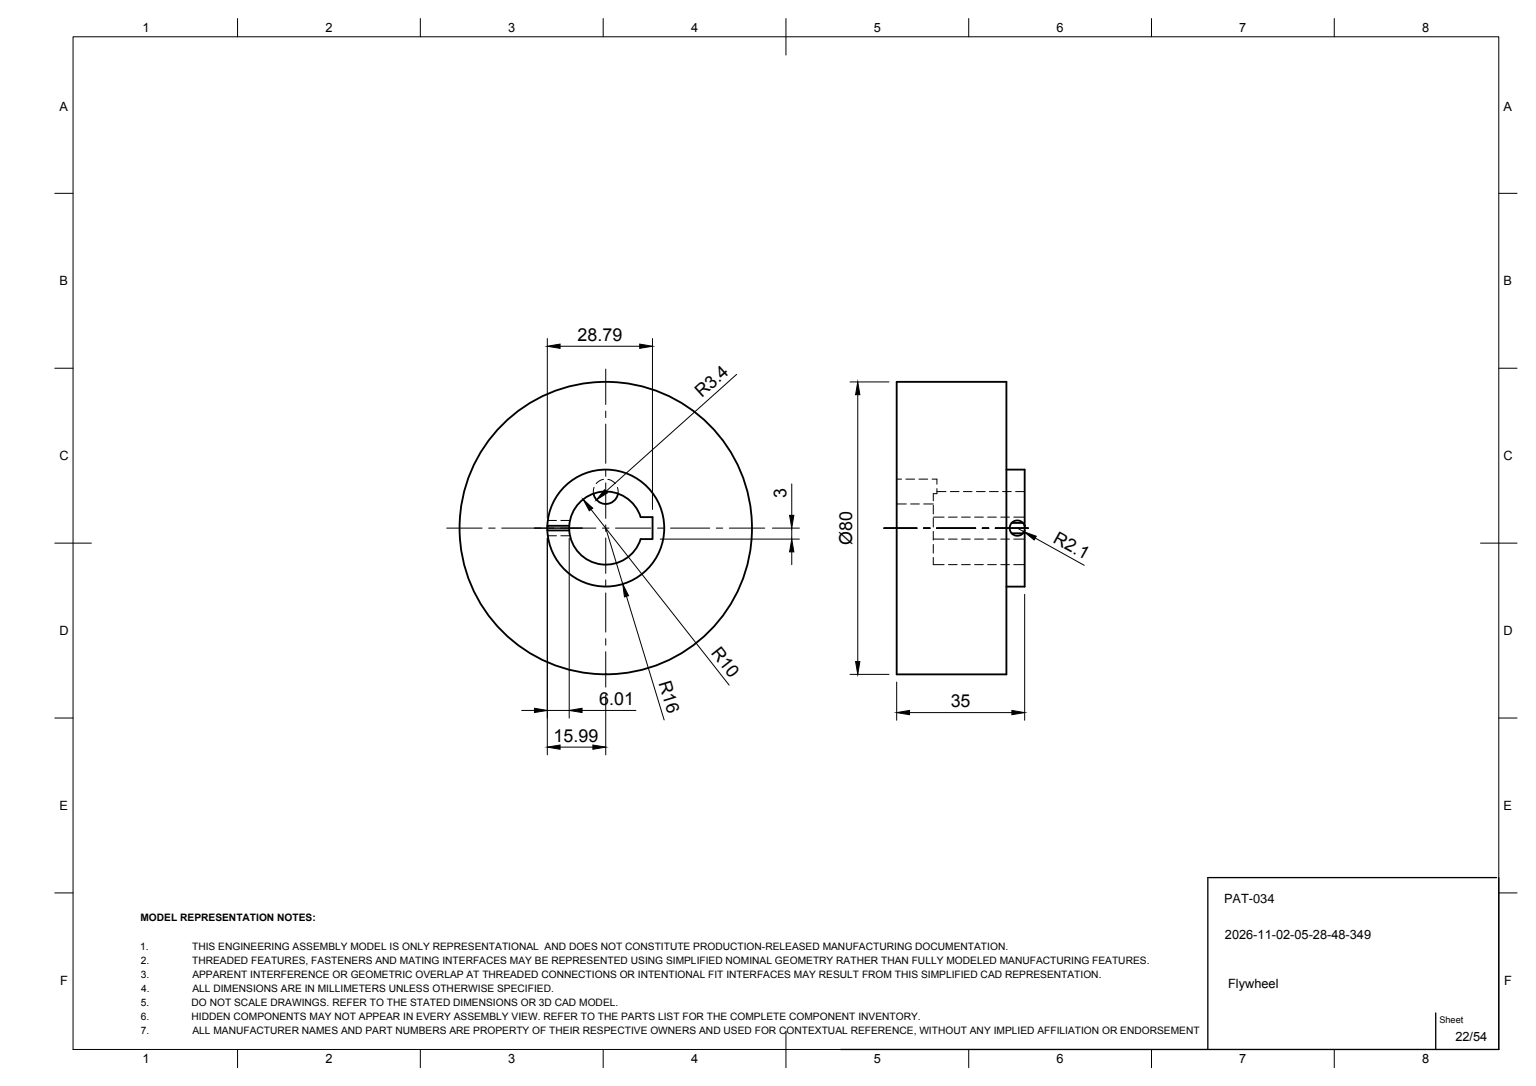
ISO-10303-21;
HEADER;
/* Generated by software containing ST-Developer
 * from STEP Tools, Inc. (www.steptools.com) 
 */

FILE_DESCRIPTION(
/* description */ ('Fatigue rig crank-slider'),
/* implementation_level */ '2;1');

FILE_NAME(
/* name */ 'Flywheel.step',
/* time_stamp */ '2026-10-28T03:24:50-07:00',
/* author */ (''),
/* organization */ (''),
/* preprocessor_version */ 'ST-DEVELOPER v20.2',
/* originating_system */ 'Autodesk Translation Framework v15.17.0.0',
/* authorisation */ '');

FILE_SCHEMA (('AUTOMOTIVE_DESIGN { 1 0 10303 214 3 1 1 }'));
ENDSEC;

DATA;
#10=MECHANICAL_DESIGN_GEOMETRIC_PRESENTATION_REPRESENTATION('',(#608),#16911);
#447=B_SPLINE_CURVE_WITH_KNOTS('',3,(#15046,#15047,#15048,#15049,#15050,
#15051),.UNSPECIFIED.,.F.,.F.,(4,2,4),(1.01510699658258,1.03166343394832,
1.10079263710785),.UNSPECIFIED.);
#448=B_SPLINE_CURVE_WITH_KNOTS('',3,(#15055,#15056,#15057,#15058,#15059,
#15060,#15061,#15062,#15063,#15064),.UNSPECIFIED.,.F.,.F.,(4,2,2,2,4),(0.168950313426779,
0.238079516586307,0.317435737633656,0.396791958681006,0.465921161840534),
 .UNSPECIFIED.);
#449=B_SPLINE_CURVE_WITH_KNOTS('',3,(#15068,#15069,#15070,#15071,#15072,
#15073),.UNSPECIFIED.,.F.,.F.,(4,2,4),(0.803821788694091,0.872950991853619,
0.88950742921936),.UNSPECIFIED.);
#450=B_SPLINE_CURVE_WITH_KNOTS('',3,(#15103,#15104,#15105,#15106,#15107,
#15108,#15109,#15110,#15111,#15112,#15113,#15114,#15115,#15116,#15117,#15118,
#15119,#15120,#15121,#15122,#15123,#15124,#15125,#15126,#15127,#15128,#15129,
#15130,#15131,#15132,#15133,#15134,#15135,#15136,#15137),.UNSPECIFIED.,
 .F.,.F.,(4,2,2,2,2,2,2,2,2,2,2,2,3,2,2,2,4),(0.379554434981269,0.396011596624156,
0.475213593758045,0.554416396369289,0.633619198980533,0.712822001591777,
0.792024804203021,0.87122680133691,0.950428798470799,1.02963079560469,1.10883279273858,
1.18803559534982,1.26723839796107,1.34644120057231,1.42564400318355,1.50484600031744,
1.52130316196033),.UNSPECIFIED.);
#507=SHAPE_REPRESENTATION_RELATIONSHIP('SRR','None',#17148,#557);
#557=ADVANCED_BREP_SHAPE_REPRESENTATION('',(#665),#16877);
#608=STYLED_ITEM('',(#17501),#665);
#665=MANIFOLD_SOLID_BREP('Body1',#8901);
#831=FACE_BOUND('',#2121,.T.);
#832=FACE_BOUND('',#2129,.T.);
#1043=PLANE('',#9952);
#1044=PLANE('',#9964);
#1045=PLANE('',#9965);
#1046=PLANE('',#9967);
#1047=PLANE('',#9968);
#1048=PLANE('',#9969);
#1049=PLANE('',#9973);
#1050=PLANE('',#9974);
#1051=PLANE('',#9975);
#1052=PLANE('',#9982);
#1462=FACE_OUTER_BOUND('',#2116,.T.);
#1463=FACE_OUTER_BOUND('',#2117,.T.);
#1464=FACE_OUTER_BOUND('',#2118,.T.);
#1465=FACE_OUTER_BOUND('',#2119,.T.);
#1466=FACE_OUTER_BOUND('',#2120,.T.);
#1467=FACE_OUTER_BOUND('',#2122,.T.);
#1468=FACE_OUTER_BOUND('',#2123,.T.);
#1469=FACE_OUTER_BOUND('',#2124,.T.);
#1470=FACE_OUTER_BOUND('',#2125,.T.);
#1471=FACE_OUTER_BOUND('',#2126,.T.);
#1472=FACE_OUTER_BOUND('',#2127,.T.);
#1473=FACE_OUTER_BOUND('',#2128,.T.);
#1474=FACE_OUTER_BOUND('',#2130,.T.);
#1475=FACE_OUTER_BOUND('',#2131,.T.);
#1476=FACE_OUTER_BOUND('',#2132,.T.);
#2116=EDGE_LOOP('',(#7026,#7027));
#2117=EDGE_LOOP('',(#7028,#7029,#7030,#7031,#7032,#7033,#7034,#7035));
#2118=EDGE_LOOP('',(#7036,#7037,#7038,#7039,#7040,#7041,#7042,#7043,#7044,
#7045,#7046,#7047,#7048,#7049));
#2119=EDGE_LOOP('',(#7050,#7051,#7052,#7053,#7054,#7055,#7056));
#2120=EDGE_LOOP('',(#7057));
#2121=EDGE_LOOP('',(#7058));
#2122=EDGE_LOOP('',(#7059,#7060,#7061,#7062));
#2123=EDGE_LOOP('',(#7063,#7064,#7065,#7066));
#2124=EDGE_LOOP('',(#7067,#7068));
#2125=EDGE_LOOP('',(#7069,#7070,#7071,#7072,#7073,#7074,#7075,#7076));
#2126=EDGE_LOOP('',(#7077,#7078));
#2127=EDGE_LOOP('',(#7079,#7080,#7081,#7082));
#2128=EDGE_LOOP('',(#7083));
#2129=EDGE_LOOP('',(#7084));
#2130=EDGE_LOOP('',(#7085,#7086,#7087,#7088));
#2131=EDGE_LOOP('',(#7089,#7090,#7091,#7092,#7093,#7094));
#2132=EDGE_LOOP('',(#7095,#7096,#7097,#7098,#7099,#7100,#7101,#7102,#7103));
#2756=LINE('',#15029,#3402);
#2757=LINE('',#15033,#3403);
#2758=LINE('',#15037,#3404);
#2759=LINE('',#15042,#3405);
#2760=LINE('',#15053,#3406);
#2761=LINE('',#15066,#3407);
#2762=LINE('',#15077,#3408);
#2763=LINE('',#15081,#3409);
#2764=LINE('',#15083,#3410);
#2765=LINE('',#15084,#3411);
#2766=LINE('',#15090,#3412);
#2767=LINE('',#15092,#3413);
#2768=LINE('',#15093,#3414);
#2769=LINE('',#15095,#3415);
#2770=LINE('',#15101,#3416);
#2771=LINE('',#15138,#3417);
#2772=LINE('',#15141,#3418);
#2773=LINE('',#15148,#3419);
#2774=LINE('',#15151,#3420);
#3402=VECTOR('',#11788,1.);
#3403=VECTOR('',#11791,0.34);
#3404=VECTOR('',#11796,1.);
#3405=VECTOR('',#11801,1.);
#3406=VECTOR('',#11804,1.);
#3407=VECTOR('',#11805,1.);
#3408=VECTOR('',#11808,1.);
#3409=VECTOR('',#11813,1.);
#3410=VECTOR('',#11814,1.);
#3411=VECTOR('',#11815,1.);
#3412=VECTOR('',#11822,1.);
#3413=VECTOR('',#11823,1.);
#3414=VECTOR('',#11824,1.);
#3415=VECTOR('',#11827,1.);
#3416=VECTOR('',#11836,1.);
#3417=VECTOR('',#11837,1.);
#3418=VECTOR('',#11842,1.);
#3419=VECTOR('',#11851,4.);
#3420=VECTOR('',#11854,1.6);
#3939=CIRCLE('',#9953,1.);
#3940=CIRCLE('',#9954,0.34);
#3941=CIRCLE('',#9956,0.34);
#3942=CIRCLE('',#9957,0.34);
#3943=CIRCLE('',#9958,0.34);
#3944=CIRCLE('',#9960,1.);
#3945=CIRCLE('',#9961,1.);
#3946=CIRCLE('',#9962,1.);
#3947=CIRCLE('',#9963,1.);
#3948=CIRCLE('',#9966,4.);
#3949=CIRCLE('',#9970,0.21);
#3950=CIRCLE('',#9972,0.21);
#3951=CIRCLE('',#9976,4.);
#3952=CIRCLE('',#9977,1.6);
#3953=CIRCLE('',#9980,1.6);
#3954=CIRCLE('',#9981,1.6);
#4501=VERTEX_POINT('',#15023);
#4502=VERTEX_POINT('',#15024);
#4503=VERTEX_POINT('',#15028);
#4504=VERTEX_POINT('',#15030);
#4505=VERTEX_POINT('',#15032);
#4506=VERTEX_POINT('',#15035);
#4507=VERTEX_POINT('',#15039);
#4508=VERTEX_POINT('',#15041);
#4509=VERTEX_POINT('',#15043);
#4510=VERTEX_POINT('',#15045);
#4511=VERTEX_POINT('',#15052);
#4512=VERTEX_POINT('',#15054);
#4513=VERTEX_POINT('',#15065);
#4514=VERTEX_POINT('',#15067);
#4515=VERTEX_POINT('',#15074);
#4516=VERTEX_POINT('',#15076);
#4517=VERTEX_POINT('',#15080);
#4518=VERTEX_POINT('',#15082);
#4519=VERTEX_POINT('',#15086);
#4520=VERTEX_POINT('',#15089);
#4521=VERTEX_POINT('',#15091);
#4522=VERTEX_POINT('',#15100);
#4523=VERTEX_POINT('',#15102);
#4524=VERTEX_POINT('',#15143);
#4525=VERTEX_POINT('',#15145);
#4526=VERTEX_POINT('',#15150);
#5411=EDGE_CURVE('',#4501,#4502,#3939,.T.);
#5412=EDGE_CURVE('',#4501,#4502,#3940,.T.);
#5413=EDGE_CURVE('',#4503,#4501,#2756,.T.);
#5414=EDGE_CURVE('',#4504,#4503,#3941,.T.);
#5415=EDGE_CURVE('',#4504,#4505,#2757,.T.);
#5416=EDGE_CURVE('',#4505,#4505,#3942,.T.);
#5417=EDGE_CURVE('',#4506,#4504,#3943,.T.);
#5418=EDGE_CURVE('',#4502,#4506,#2758,.T.);
#5419=EDGE_CURVE('',#4506,#4507,#3944,.T.);
#5420=EDGE_CURVE('',#4507,#4508,#2759,.T.);
#5421=EDGE_CURVE('',#4508,#4509,#3945,.T.);
#5422=EDGE_CURVE('',#4509,#4510,#447,.T.);
#5423=EDGE_CURVE('',#4510,#4511,#2760,.T.);
#5424=EDGE_CURVE('',#4511,#4512,#448,.T.);
#5425=EDGE_CURVE('',#4512,#4513,#2761,.T.);
#5426=EDGE_CURVE('',#4513,#4514,#449,.T.);
#5427=EDGE_CURVE('',#4514,#4515,#3946,.T.);
#5428=EDGE_CURVE('',#4515,#4516,#2762,.T.);
#5429=EDGE_CURVE('',#4516,#4503,#3947,.T.);
#5430=EDGE_CURVE('',#4517,#4516,#2763,.T.);
#5431=EDGE_CURVE('',#4518,#4517,#2764,.T.);
#5432=EDGE_CURVE('',#4507,#4518,#2765,.T.);
#5433=EDGE_CURVE('',#4519,#4519,#3948,.T.);
#5434=EDGE_CURVE('',#4520,#4517,#2766,.T.);
#5435=EDGE_CURVE('',#4521,#4520,#2767,.T.);
#5436=EDGE_CURVE('',#4521,#4518,#2768,.T.);
#5437=EDGE_CURVE('',#4520,#4515,#2769,.T.);
#5438=EDGE_CURVE('',#4512,#4513,#3949,.T.);
#5439=EDGE_CURVE('',#4510,#4511,#3950,.T.);
#5440=EDGE_CURVE('',#4522,#4509,#2770,.T.);
#5441=EDGE_CURVE('',#4523,#4522,#450,.T.);
#5442=EDGE_CURVE('',#4514,#4523,#2771,.T.);
#5443=EDGE_CURVE('',#4508,#4521,#2772,.T.);
#5444=EDGE_CURVE('',#4524,#4524,#3951,.T.);
#5445=EDGE_CURVE('',#4525,#4525,#3952,.T.);
#5446=EDGE_CURVE('',#4519,#4524,#2773,.T.);
#5447=EDGE_CURVE('',#4525,#4526,#2774,.T.);
#5448=EDGE_CURVE('',#4526,#4523,#3953,.T.);
#5449=EDGE_CURVE('',#4522,#4526,#3954,.T.);
#7026=ORIENTED_EDGE('',*,*,#5411,.F.);
#7027=ORIENTED_EDGE('',*,*,#5412,.T.);
#7028=ORIENTED_EDGE('',*,*,#5413,.F.);
#7029=ORIENTED_EDGE('',*,*,#5414,.F.);
#7030=ORIENTED_EDGE('',*,*,#5415,.T.);
#7031=ORIENTED_EDGE('',*,*,#5416,.F.);
#7032=ORIENTED_EDGE('',*,*,#5415,.F.);
#7033=ORIENTED_EDGE('',*,*,#5417,.F.);
#7034=ORIENTED_EDGE('',*,*,#5418,.F.);
#7035=ORIENTED_EDGE('',*,*,#5412,.F.);
#7036=ORIENTED_EDGE('',*,*,#5413,.T.);
#7037=ORIENTED_EDGE('',*,*,#5411,.T.);
#7038=ORIENTED_EDGE('',*,*,#5418,.T.);
#7039=ORIENTED_EDGE('',*,*,#5419,.T.);
#7040=ORIENTED_EDGE('',*,*,#5420,.T.);
#7041=ORIENTED_EDGE('',*,*,#5421,.T.);
#7042=ORIENTED_EDGE('',*,*,#5422,.T.);
#7043=ORIENTED_EDGE('',*,*,#5423,.T.);
#7044=ORIENTED_EDGE('',*,*,#5424,.T.);
#7045=ORIENTED_EDGE('',*,*,#5425,.T.);
#7046=ORIENTED_EDGE('',*,*,#5426,.T.);
#7047=ORIENTED_EDGE('',*,*,#5427,.T.);
#7048=ORIENTED_EDGE('',*,*,#5428,.T.);
#7049=ORIENTED_EDGE('',*,*,#5429,.T.);
#7050=ORIENTED_EDGE('',*,*,#5417,.T.);
#7051=ORIENTED_EDGE('',*,*,#5414,.T.);
#7052=ORIENTED_EDGE('',*,*,#5429,.F.);
#7053=ORIENTED_EDGE('',*,*,#5430,.F.);
#7054=ORIENTED_EDGE('',*,*,#5431,.F.);
#7055=ORIENTED_EDGE('',*,*,#5432,.F.);
#7056=ORIENTED_EDGE('',*,*,#5419,.F.);
#7057=ORIENTED_EDGE('',*,*,#5433,.T.);
#7058=ORIENTED_EDGE('',*,*,#5416,.T.);
#7059=ORIENTED_EDGE('',*,*,#5431,.T.);
#7060=ORIENTED_EDGE('',*,*,#5434,.F.);
#7061=ORIENTED_EDGE('',*,*,#5435,.F.);
#7062=ORIENTED_EDGE('',*,*,#5436,.T.);
#7063=ORIENTED_EDGE('',*,*,#5430,.T.);
#7064=ORIENTED_EDGE('',*,*,#5428,.F.);
#7065=ORIENTED_EDGE('',*,*,#5437,.F.);
#7066=ORIENTED_EDGE('',*,*,#5434,.T.);
#7067=ORIENTED_EDGE('',*,*,#5425,.F.);
#7068=ORIENTED_EDGE('',*,*,#5438,.T.);
#7069=ORIENTED_EDGE('',*,*,#5424,.F.);
#7070=ORIENTED_EDGE('',*,*,#5439,.F.);
#7071=ORIENTED_EDGE('',*,*,#5422,.F.);
#7072=ORIENTED_EDGE('',*,*,#5440,.F.);
#7073=ORIENTED_EDGE('',*,*,#5441,.F.);
#7074=ORIENTED_EDGE('',*,*,#5442,.F.);
#7075=ORIENTED_EDGE('',*,*,#5426,.F.);
#7076=ORIENTED_EDGE('',*,*,#5438,.F.);
#7077=ORIENTED_EDGE('',*,*,#5423,.F.);
#7078=ORIENTED_EDGE('',*,*,#5439,.T.);
#7079=ORIENTED_EDGE('',*,*,#5432,.T.);
#7080=ORIENTED_EDGE('',*,*,#5436,.F.);
#7081=ORIENTED_EDGE('',*,*,#5443,.F.);
#7082=ORIENTED_EDGE('',*,*,#5420,.F.);
#7083=ORIENTED_EDGE('',*,*,#5444,.F.);
#7084=ORIENTED_EDGE('',*,*,#5445,.F.);
#7085=ORIENTED_EDGE('',*,*,#5433,.F.);
#7086=ORIENTED_EDGE('',*,*,#5446,.T.);
#7087=ORIENTED_EDGE('',*,*,#5444,.T.);
#7088=ORIENTED_EDGE('',*,*,#5446,.F.);
#7089=ORIENTED_EDGE('',*,*,#5445,.T.);
#7090=ORIENTED_EDGE('',*,*,#5447,.T.);
#7091=ORIENTED_EDGE('',*,*,#5448,.T.);
#7092=ORIENTED_EDGE('',*,*,#5441,.T.);
#7093=ORIENTED_EDGE('',*,*,#5449,.T.);
#7094=ORIENTED_EDGE('',*,*,#5447,.F.);
#7095=ORIENTED_EDGE('',*,*,#5440,.T.);
#7096=ORIENTED_EDGE('',*,*,#5421,.F.);
#7097=ORIENTED_EDGE('',*,*,#5443,.T.);
#7098=ORIENTED_EDGE('',*,*,#5435,.T.);
#7099=ORIENTED_EDGE('',*,*,#5437,.T.);
#7100=ORIENTED_EDGE('',*,*,#5427,.F.);
#7101=ORIENTED_EDGE('',*,*,#5442,.T.);
#7102=ORIENTED_EDGE('',*,*,#5448,.F.);
#7103=ORIENTED_EDGE('',*,*,#5449,.F.);
#8286=CYLINDRICAL_SURFACE('',#9955,0.34);
#8287=CYLINDRICAL_SURFACE('',#9959,1.);
#8288=CYLINDRICAL_SURFACE('',#9971,0.21);
#8289=CYLINDRICAL_SURFACE('',#9978,4.);
#8290=CYLINDRICAL_SURFACE('',#9979,1.6);
#8600=ADVANCED_FACE('',(#1462),#1043,.T.);
#8601=ADVANCED_FACE('',(#1463),#8286,.F.);
#8602=ADVANCED_FACE('',(#1464),#8287,.F.);
#8603=ADVANCED_FACE('',(#1465),#1044,.F.);
#8604=ADVANCED_FACE('',(#1466,#831),#1045,.T.);
#8605=ADVANCED_FACE('',(#1467),#1046,.F.);
#8606=ADVANCED_FACE('',(#1468),#1047,.F.);
#8607=ADVANCED_FACE('',(#1469),#1048,.T.);
#8608=ADVANCED_FACE('',(#1470),#8288,.F.);
#8609=ADVANCED_FACE('',(#1471),#1049,.T.);
#8610=ADVANCED_FACE('',(#1472),#1050,.F.);
#8611=ADVANCED_FACE('',(#1473,#832),#1051,.F.);
#8612=ADVANCED_FACE('',(#1474),#8289,.T.);
#8613=ADVANCED_FACE('',(#1475),#8290,.T.);
#8614=ADVANCED_FACE('',(#1476),#1052,.F.);
#8901=CLOSED_SHELL('',(#8600,#8601,#8602,#8603,#8604,#8605,#8606,#8607,
#8608,#8609,#8610,#8611,#8612,#8613,#8614));
#9951=AXIS2_PLACEMENT_3D('',#15021,#11778,#11779);
#9952=AXIS2_PLACEMENT_3D('',#15022,#11780,#11781);
#9953=AXIS2_PLACEMENT_3D('',#15025,#11782,#11783);
#9954=AXIS2_PLACEMENT_3D('',#15026,#11784,#11785);
#9955=AXIS2_PLACEMENT_3D('',#15027,#11786,#11787);
#9956=AXIS2_PLACEMENT_3D('',#15031,#11789,#11790);
#9957=AXIS2_PLACEMENT_3D('',#15034,#11792,#11793);
#9958=AXIS2_PLACEMENT_3D('',#15036,#11794,#11795);
#9959=AXIS2_PLACEMENT_3D('',#15038,#11797,#11798);
#9960=AXIS2_PLACEMENT_3D('',#15040,#11799,#11800);
#9961=AXIS2_PLACEMENT_3D('',#15044,#11802,#11803);
#9962=AXIS2_PLACEMENT_3D('',#15075,#11806,#11807);
#9963=AXIS2_PLACEMENT_3D('',#15078,#11809,#11810);
#9964=AXIS2_PLACEMENT_3D('',#15079,#11811,#11812);
#9965=AXIS2_PLACEMENT_3D('',#15085,#11816,#11817);
#9966=AXIS2_PLACEMENT_3D('',#15087,#11818,#11819);
#9967=AXIS2_PLACEMENT_3D('',#15088,#11820,#11821);
#9968=AXIS2_PLACEMENT_3D('',#15094,#11825,#11826);
#9969=AXIS2_PLACEMENT_3D('',#15096,#11828,#11829);
#9970=AXIS2_PLACEMENT_3D('',#15097,#11830,#11831);
#9971=AXIS2_PLACEMENT_3D('',#15098,#11832,#11833);
#9972=AXIS2_PLACEMENT_3D('',#15099,#11834,#11835);
#9973=AXIS2_PLACEMENT_3D('',#15139,#11838,#11839);
#9974=AXIS2_PLACEMENT_3D('',#15140,#11840,#11841);
#9975=AXIS2_PLACEMENT_3D('',#15142,#11843,#11844);
#9976=AXIS2_PLACEMENT_3D('',#15144,#11845,#11846);
#9977=AXIS2_PLACEMENT_3D('',#15146,#11847,#11848);
#9978=AXIS2_PLACEMENT_3D('',#15147,#11849,#11850);
#9979=AXIS2_PLACEMENT_3D('',#15149,#11852,#11853);
#9980=AXIS2_PLACEMENT_3D('',#15152,#11855,#11856);
#9981=AXIS2_PLACEMENT_3D('',#15153,#11857,#11858);
#9982=AXIS2_PLACEMENT_3D('',#15154,#11859,#11860);
#11778=DIRECTION('axis',(0.,0.,1.));
#11779=DIRECTION('refdir',(1.,0.,0.));
#11780=DIRECTION('center_axis',(0.,1.,0.));
#11781=DIRECTION('ref_axis',(1.,0.,0.));
#11782=DIRECTION('center_axis',(0.,1.,0.));
#11783=DIRECTION('ref_axis',(1.,0.,0.));
#11784=DIRECTION('center_axis',(0.,1.,0.));
#11785=DIRECTION('ref_axis',(1.,0.,0.));
#11786=DIRECTION('center_axis',(0.,1.,0.));
#11787=DIRECTION('ref_axis',(1.,0.,0.));
#11788=DIRECTION('',(0.,-1.,0.));
#11789=DIRECTION('center_axis',(0.,1.,0.));
#11790=DIRECTION('ref_axis',(1.,0.,0.));
#11791=DIRECTION('',(0.,1.,0.));
#11792=DIRECTION('center_axis',(0.,-1.,0.));
#11793=DIRECTION('ref_axis',(1.,0.,0.));
#11794=DIRECTION('center_axis',(0.,1.,0.));
#11795=DIRECTION('ref_axis',(1.,0.,0.));
#11796=DIRECTION('',(0.,1.,0.));
#11797=DIRECTION('center_axis',(0.,1.,0.));
#11798=DIRECTION('ref_axis',(6.12323399573677E-17,0.,1.));
#11799=DIRECTION('center_axis',(0.,1.,0.));
#11800=DIRECTION('ref_axis',(1.,0.,0.));
#11801=DIRECTION('',(0.,-1.,0.));
#11802=DIRECTION('center_axis',(0.,-1.,0.));
#11803=DIRECTION('ref_axis',(1.,0.,0.));
#11804=DIRECTION('',(0.,1.,0.));
#11805=DIRECTION('',(0.,-1.,0.));
#11806=DIRECTION('center_axis',(0.,-1.,0.));
#11807=DIRECTION('ref_axis',(1.,0.,0.));
#11808=DIRECTION('',(0.,1.,0.));
#11809=DIRECTION('center_axis',(0.,1.,0.));
#11810=DIRECTION('ref_axis',(1.,0.,0.));
#11811=DIRECTION('center_axis',(0.,1.,0.));
#11812=DIRECTION('ref_axis',(1.,0.,0.));
#11813=DIRECTION('',(0.,0.,1.));
#11814=DIRECTION('',(-1.,0.,0.));
#11815=DIRECTION('',(0.,0.,-1.));
#11816=DIRECTION('center_axis',(0.,1.,0.));
#11817=DIRECTION('ref_axis',(1.,0.,0.));
#11818=DIRECTION('center_axis',(0.,1.,0.));
#11819=DIRECTION('ref_axis',(1.,0.,0.));
#11820=DIRECTION('center_axis',(0.,0.,-1.));
#11821=DIRECTION('ref_axis',(-1.,0.,0.));
#11822=DIRECTION('',(0.,1.,0.));
#11823=DIRECTION('',(-1.,0.,0.));
#11824=DIRECTION('',(0.,1.,0.));
#11825=DIRECTION('center_axis',(-1.,0.,0.));
#11826=DIRECTION('ref_axis',(0.,0.,1.));
#11827=DIRECTION('',(0.,0.,1.));
#11828=DIRECTION('center_axis',(0.,0.,1.));
#11829=DIRECTION('ref_axis',(1.,0.,0.));
#11830=DIRECTION('center_axis',(0.,0.,1.));
#11831=DIRECTION('ref_axis',(1.,0.,0.));
#11832=DIRECTION('center_axis',(0.,0.,1.));
#11833=DIRECTION('ref_axis',(6.12323399573677E-17,1.,0.));
#11834=DIRECTION('center_axis',(0.,0.,1.));
#11835=DIRECTION('ref_axis',(1.,0.,0.));
#11836=DIRECTION('',(0.,0.,-1.));
#11837=DIRECTION('',(0.,0.,1.));
#11838=DIRECTION('center_axis',(0.,0.,1.));
#11839=DIRECTION('ref_axis',(1.,0.,0.));
#11840=DIRECTION('center_axis',(1.,0.,0.));
#11841=DIRECTION('ref_axis',(0.,0.,-1.));
#11842=DIRECTION('',(0.,0.,-1.));
#11843=DIRECTION('center_axis',(0.,1.,0.));
#11844=DIRECTION('ref_axis',(1.,0.,0.));
#11845=DIRECTION('center_axis',(0.,1.,0.));
#11846=DIRECTION('ref_axis',(1.,0.,0.));
#11847=DIRECTION('center_axis',(0.,-1.,0.));
#11848=DIRECTION('ref_axis',(1.,0.,0.));
#11849=DIRECTION('center_axis',(0.,1.,0.));
#11850=DIRECTION('ref_axis',(1.,0.,0.));
#11851=DIRECTION('',(0.,-1.,0.));
#11852=DIRECTION('center_axis',(0.,1.,0.));
#11853=DIRECTION('ref_axis',(1.,0.,0.));
#11854=DIRECTION('',(0.,-1.,0.));
#11855=DIRECTION('center_axis',(0.,1.,0.));
#11856=DIRECTION('ref_axis',(1.,0.,0.));
#11857=DIRECTION('center_axis',(0.,1.,0.));
#11858=DIRECTION('ref_axis',(1.,0.,0.));
#11859=DIRECTION('center_axis',(0.,1.,0.));
#11860=DIRECTION('ref_axis',(1.,0.,0.));
#15021=CARTESIAN_POINT('',(0.,0.,0.));
#15022=CARTESIAN_POINT('Origin',(1.,0.9,12.));
#15023=CARTESIAN_POINT('',(0.9422,0.9,12.3350509811954));
#15024=CARTESIAN_POINT('',(0.9422,0.9,11.6649490188046));
#15025=CARTESIAN_POINT('Origin',(0.,0.9,12.));
#15026=CARTESIAN_POINT('Origin',(1.,0.9,12.));
#15027=CARTESIAN_POINT('Origin',(1.,0.9,12.));
#15028=CARTESIAN_POINT('',(0.9422,1.,12.3350509811954));
#15029=CARTESIAN_POINT('',(0.9422,0.9,12.3350509811954));
#15030=CARTESIAN_POINT('',(0.66,1.,12.));
#15031=CARTESIAN_POINT('Origin',(1.,1.,12.));
#15032=CARTESIAN_POINT('',(0.66,2.,12.));
#15033=CARTESIAN_POINT('',(0.66,0.9,12.));
#15034=CARTESIAN_POINT('Origin',(1.,2.,12.));
#15035=CARTESIAN_POINT('',(0.9422,1.,11.6649490188046));
#15036=CARTESIAN_POINT('Origin',(1.,1.,12.));
#15037=CARTESIAN_POINT('',(0.9422,0.9,11.6649490188046));
#15038=CARTESIAN_POINT('Origin',(0.,-1.5,12.));
#15039=CARTESIAN_POINT('',(0.3,1.,11.0460607985831));
#15040=CARTESIAN_POINT('Origin',(0.,1.,12.));
#15041=CARTESIAN_POINT('',(0.3,-1.5,11.0460607985831));
#15042=CARTESIAN_POINT('',(0.3,-1.5,11.0460607985831));
#15043=CARTESIAN_POINT('',(0.0640312423743287,-1.5,12.9979478944314));
#15044=CARTESIAN_POINT('Origin',(0.,-1.5,12.));
#15045=CARTESIAN_POINT('',(0.141067359796645,-1.45556349186105,12.99));
#15046=CARTESIAN_POINT('Ctrl Pts',(0.0640312423743286,-1.5,12.9979478944314));
#15047=CARTESIAN_POINT('Ctrl Pts',(0.069586383475953,-1.49822148706849,
12.9975914604048));
#15048=CARTESIAN_POINT('Ctrl Pts',(0.0750776578932034,-1.49620769804413,
12.9971923790166));
#15049=CARTESIAN_POINT('Ctrl Pts',(0.102998643109694,-1.48462404333102,
12.9949381930495));
#15050=CARTESIAN_POINT('Ctrl Pts',(0.123818356698215,-1.4712051523632,12.9924578498245));
#15051=CARTESIAN_POINT('Ctrl Pts',(0.141067359796645,-1.45556349186105,
12.99));
#15052=CARTESIAN_POINT('',(0.141067359796645,-1.14443650813895,12.99));
#15053=CARTESIAN_POINT('',(0.141067359796645,-1.5,12.99));
#15054=CARTESIAN_POINT('',(-0.141067359796645,-1.14443650813895,12.99));
#15055=CARTESIAN_POINT('Ctrl Pts',(0.141067359796645,-1.14443650813895,
12.99));
#15056=CARTESIAN_POINT('Ctrl Pts',(0.123818356698214,-1.1287948476368,12.9924578498245));
#15057=CARTESIAN_POINT('Ctrl Pts',(0.102998643109694,-1.11537595666898,
12.9949381930495));
#15058=CARTESIAN_POINT('Ctrl Pts',(0.054614114398353,-1.09530253627557,
12.9988444923724));
#15059=CARTESIAN_POINT('Ctrl Pts',(0.0264520736824499,-1.09,13.));
#15060=CARTESIAN_POINT('Ctrl Pts',(-0.0264520736824498,-1.09,13.));
#15061=CARTESIAN_POINT('Ctrl Pts',(-0.0546141143983528,-1.09530253627557,
12.9988444923724));
#15062=CARTESIAN_POINT('Ctrl Pts',(-0.102998643109694,-1.11537595666898,
12.9949381930495));
#15063=CARTESIAN_POINT('Ctrl Pts',(-0.123818356698214,-1.1287948476368,
12.9924578498245));
#15064=CARTESIAN_POINT('Ctrl Pts',(-0.141067359796645,-1.14443650813895,
12.99));
#15065=CARTESIAN_POINT('',(-0.141067359796645,-1.45556349186105,12.99));
#15066=CARTESIAN_POINT('',(-0.141067359796645,-1.5,12.99));
#15067=CARTESIAN_POINT('',(-0.0640312423743287,-1.5,12.9979478944314));
#15068=CARTESIAN_POINT('Ctrl Pts',(-0.141067359796645,-1.45556349186105,
12.99));
#15069=CARTESIAN_POINT('Ctrl Pts',(-0.123818356698214,-1.4712051523632,
12.9924578498245));
#15070=CARTESIAN_POINT('Ctrl Pts',(-0.102998643109694,-1.48462404333102,
12.9949381930495));
#15071=CARTESIAN_POINT('Ctrl Pts',(-0.0750776578932035,-1.49620769804413,
12.9971923790166));
#15072=CARTESIAN_POINT('Ctrl Pts',(-0.0695863834759529,-1.49822148706849,
12.9975914604048));
#15073=CARTESIAN_POINT('Ctrl Pts',(-0.0640312423743286,-1.5,12.9979478944314));
#15074=CARTESIAN_POINT('',(-0.3,-1.5,11.0460607985831));
#15075=CARTESIAN_POINT('Origin',(0.,-1.5,12.));
#15076=CARTESIAN_POINT('',(-0.3,1.,11.0460607985831));
#15077=CARTESIAN_POINT('',(-0.3,-1.5,11.0460607985831));
#15078=CARTESIAN_POINT('Origin',(0.,1.,12.));
#15079=CARTESIAN_POINT('Origin',(0.,1.,12.));
#15080=CARTESIAN_POINT('',(-0.3,1.,10.72));
#15081=CARTESIAN_POINT('',(-0.3,1.,11.36));
#15082=CARTESIAN_POINT('',(0.3,1.,10.72));
#15083=CARTESIAN_POINT('',(0.15,1.,10.72));
#15084=CARTESIAN_POINT('',(0.3,1.,12.));
#15085=CARTESIAN_POINT('Origin',(0.,2.,12.));
#15086=CARTESIAN_POINT('',(-4.,2.,12.));
#15087=CARTESIAN_POINT('Origin',(0.,2.,12.));
#15088=CARTESIAN_POINT('Origin',(0.3,-1.6,10.72));
#15089=CARTESIAN_POINT('',(-0.3,-1.5,10.72));
#15090=CARTESIAN_POINT('',(-0.3,-1.6,10.72));
#15091=CARTESIAN_POINT('',(0.3,-1.5,10.72));
#15092=CARTESIAN_POINT('',(0.15,-1.5,10.72));
#15093=CARTESIAN_POINT('',(0.3,-1.6,10.72));
#15094=CARTESIAN_POINT('Origin',(-0.3,-1.6,10.72));
#15095=CARTESIAN_POINT('',(-0.3,-1.5,11.36));
#15096=CARTESIAN_POINT('Origin',(0.,-1.3,12.99));
#15097=CARTESIAN_POINT('Origin',(0.,-1.3,12.99));
#15098=CARTESIAN_POINT('Origin',(0.,-1.3,12.99));
#15099=CARTESIAN_POINT('Origin',(0.,-1.3,12.99));
#15100=CARTESIAN_POINT('',(0.0640312423743287,-1.5,13.5987182365883));
#15101=CARTESIAN_POINT('',(0.0640312423743287,-1.5,12.99));
#15102=CARTESIAN_POINT('',(-0.0640312423743287,-1.5,13.5987182365883));
#15103=CARTESIAN_POINT('Ctrl Pts',(-0.0640312423743288,-1.5,13.5987182365883));
#15104=CARTESIAN_POINT('Ctrl Pts',(-0.0695623721690264,-1.49822917443756,
13.5984967059243));
#15105=CARTESIAN_POINT('Ctrl Pts',(-0.0750312749053374,-1.49622475645458,
13.5982488123351));
#15106=CARTESIAN_POINT('Ctrl Pts',(-0.106271159541076,-1.48327680083123,
13.5966769093301));
#15107=CARTESIAN_POINT('Ctrl Pts',(-0.129864750292352,-1.467120097806,13.5948307595328));
#15108=CARTESIAN_POINT('Ctrl Pts',(-0.167120287247804,-1.42986456085055,
13.5913581688701));
#15109=CARTESIAN_POINT('Ctrl Pts',(-0.183276841782292,-1.4062710523005,
13.5895050296478));
#15110=CARTESIAN_POINT('Ctrl Pts',(-0.20471752266132,-1.35454055536511,
13.586886062954));
#15111=CARTESIAN_POINT('Ctrl Pts',(-0.21,-1.32640093420375,13.5861588823318));
#15112=CARTESIAN_POINT('Ctrl Pts',(-0.21,-1.27359906579625,13.5861588823318));
#15113=CARTESIAN_POINT('Ctrl Pts',(-0.20471752266132,-1.24545944463489,
13.586886062954));
#15114=CARTESIAN_POINT('Ctrl Pts',(-0.183276841782292,-1.1937289476995,
13.5895050296478));
#15115=CARTESIAN_POINT('Ctrl Pts',(-0.167120287247804,-1.17013543914945,
13.5913581688701));
#15116=CARTESIAN_POINT('Ctrl Pts',(-0.129864750292352,-1.132879902194,13.5948307595328));
#15117=CARTESIAN_POINT('Ctrl Pts',(-0.106271159541076,-1.11672319916877,
13.5966769093301));
#15118=CARTESIAN_POINT('Ctrl Pts',(-0.0545403836274686,-1.0952824096556,
13.5992798562698));
#15119=CARTESIAN_POINT('Ctrl Pts',(-0.0264006657112965,-1.09,13.6));
#15120=CARTESIAN_POINT('Ctrl Pts',(0.0264006657112964,-1.09,13.6));
#15121=CARTESIAN_POINT('Ctrl Pts',(0.0545403836274687,-1.0952824096556,
13.5992798562698));
#15122=CARTESIAN_POINT('Ctrl Pts',(0.106271159541076,-1.11672319916877,
13.5966769093301));
#15123=CARTESIAN_POINT('Ctrl Pts',(0.129864750292352,-1.132879902194,13.5948307595328));
#15124=CARTESIAN_POINT('Ctrl Pts',(0.167120287247804,-1.17013543914945,
13.5913581688701));
#15125=CARTESIAN_POINT('Ctrl Pts',(0.183276841782292,-1.1937289476995,13.5895050296478));
#15126=CARTESIAN_POINT('Ctrl Pts',(0.20471752266132,-1.24545944463489,13.586886062954));
#15127=CARTESIAN_POINT('Ctrl Pts',(0.21,-1.27359906579625,13.5861588823318));
#15128=CARTESIAN_POINT('Ctrl Pts',(0.21,-1.3,13.5861588823318));
#15129=CARTESIAN_POINT('Ctrl Pts',(0.21,-1.32640093420375,13.5861588823318));
#15130=CARTESIAN_POINT('Ctrl Pts',(0.20471752266132,-1.35454055536511,13.586886062954));
#15131=CARTESIAN_POINT('Ctrl Pts',(0.183276841782292,-1.4062710523005,13.5895050296478));
#15132=CARTESIAN_POINT('Ctrl Pts',(0.167120287247804,-1.42986456085055,
13.5913581688701));
#15133=CARTESIAN_POINT('Ctrl Pts',(0.129864750292352,-1.467120097806,13.5948307595328));
#15134=CARTESIAN_POINT('Ctrl Pts',(0.106271159541076,-1.48327680083123,
13.5966769093301));
#15135=CARTESIAN_POINT('Ctrl Pts',(0.0750312749053373,-1.49622475645458,
13.5982488123351));
#15136=CARTESIAN_POINT('Ctrl Pts',(0.0695623721690265,-1.49822917443756,
13.5984967059243));
#15137=CARTESIAN_POINT('Ctrl Pts',(0.0640312423743287,-1.5,13.5987182365883));
#15138=CARTESIAN_POINT('',(-0.0640312423743287,-1.5,12.99));
#15139=CARTESIAN_POINT('Origin',(0.,-1.3,12.99));
#15140=CARTESIAN_POINT('Origin',(0.3,-1.6,12.));
#15141=CARTESIAN_POINT('',(0.3,-1.5,12.));
#15142=CARTESIAN_POINT('Origin',(0.,-1.,12.));
#15143=CARTESIAN_POINT('',(-4.,-1.,12.));
#15144=CARTESIAN_POINT('Origin',(0.,-1.,12.));
#15145=CARTESIAN_POINT('',(-1.6,-1.,12.));
#15146=CARTESIAN_POINT('Origin',(0.,-1.,12.));
#15147=CARTESIAN_POINT('Origin',(0.,-1.,12.));
#15148=CARTESIAN_POINT('',(-4.,-1.,12.));
#15149=CARTESIAN_POINT('Origin',(0.,-1.5,12.));
#15150=CARTESIAN_POINT('',(-1.6,-1.5,12.));
#15151=CARTESIAN_POINT('',(-1.6,-1.5,12.));
#15152=CARTESIAN_POINT('Origin',(0.,-1.5,12.));
#15153=CARTESIAN_POINT('Origin',(0.,-1.5,12.));
#15154=CARTESIAN_POINT('Origin',(0.,-1.5,12.));
#16818=UNCERTAINTY_MEASURE_WITH_UNIT(LENGTH_MEASURE(0.001),#16912,
'DISTANCE_ACCURACY_VALUE',
'Maximum model space distance between geometric entities at asserted c
onnectivities');
#16852=UNCERTAINTY_MEASURE_WITH_UNIT(LENGTH_MEASURE(0.001),#16912,
'DISTANCE_ACCURACY_VALUE',
'Maximum model space distance between geometric entities at asserted c
onnectivities');
#16877=(
GEOMETRIC_REPRESENTATION_CONTEXT(3)
GLOBAL_UNCERTAINTY_ASSIGNED_CONTEXT((#16818))
GLOBAL_UNIT_ASSIGNED_CONTEXT((#16912,#16914,#16915))
REPRESENTATION_CONTEXT('','3D')
);
#16911=(
GEOMETRIC_REPRESENTATION_CONTEXT(3)
GLOBAL_UNCERTAINTY_ASSIGNED_CONTEXT((#16852))
GLOBAL_UNIT_ASSIGNED_CONTEXT((#16912,#16914,#16915))
REPRESENTATION_CONTEXT('','3D')
);
#16912=(
LENGTH_UNIT()
NAMED_UNIT(*)
SI_UNIT(.CENTI.,.METRE.)
);
#16914=(
NAMED_UNIT(*)
PLANE_ANGLE_UNIT()
SI_UNIT($,.RADIAN.)
);
#16915=(
NAMED_UNIT(*)
SI_UNIT($,.STERADIAN.)
SOLID_ANGLE_UNIT()
);
#16940=SHAPE_DEFINITION_REPRESENTATION(#17000,#17148);
#17000=PRODUCT_DEFINITION_SHAPE('',$,#17207);
#17148=SHAPE_REPRESENTATION('',(#9951),#16877);
#17182=PRODUCT_DEFINITION_CONTEXT('part definition',#17358,'design');
#17207=PRODUCT_DEFINITION('Flywheel','Flywheel',#17265,#17182);
#17265=PRODUCT_DEFINITION_FORMATION('',$,#17384);
#17358=APPLICATION_CONTEXT(
'Core Data for Automotive Mechanical Design Process');
#17359=PRODUCT_CONTEXT('part definition',#17358,'mechanical');
#17384=PRODUCT('Flywheel','Flywheel','Flywheel',(#17359));
#17495=COLOUR_RGB('Off White',0.89,0.88,0.83);
#17496=FILL_AREA_STYLE_COLOUR('',#17495);
#17497=FILL_AREA_STYLE('',(#17496));
#17498=SURFACE_STYLE_FILL_AREA(#17497);
#17499=SURFACE_SIDE_STYLE('',(#17498));
#17500=SURFACE_STYLE_USAGE(.BOTH.,#17499);
#17501=PRESENTATION_STYLE_ASSIGNMENT((#17500));
ENDSEC;
END-ISO-10303-21;
